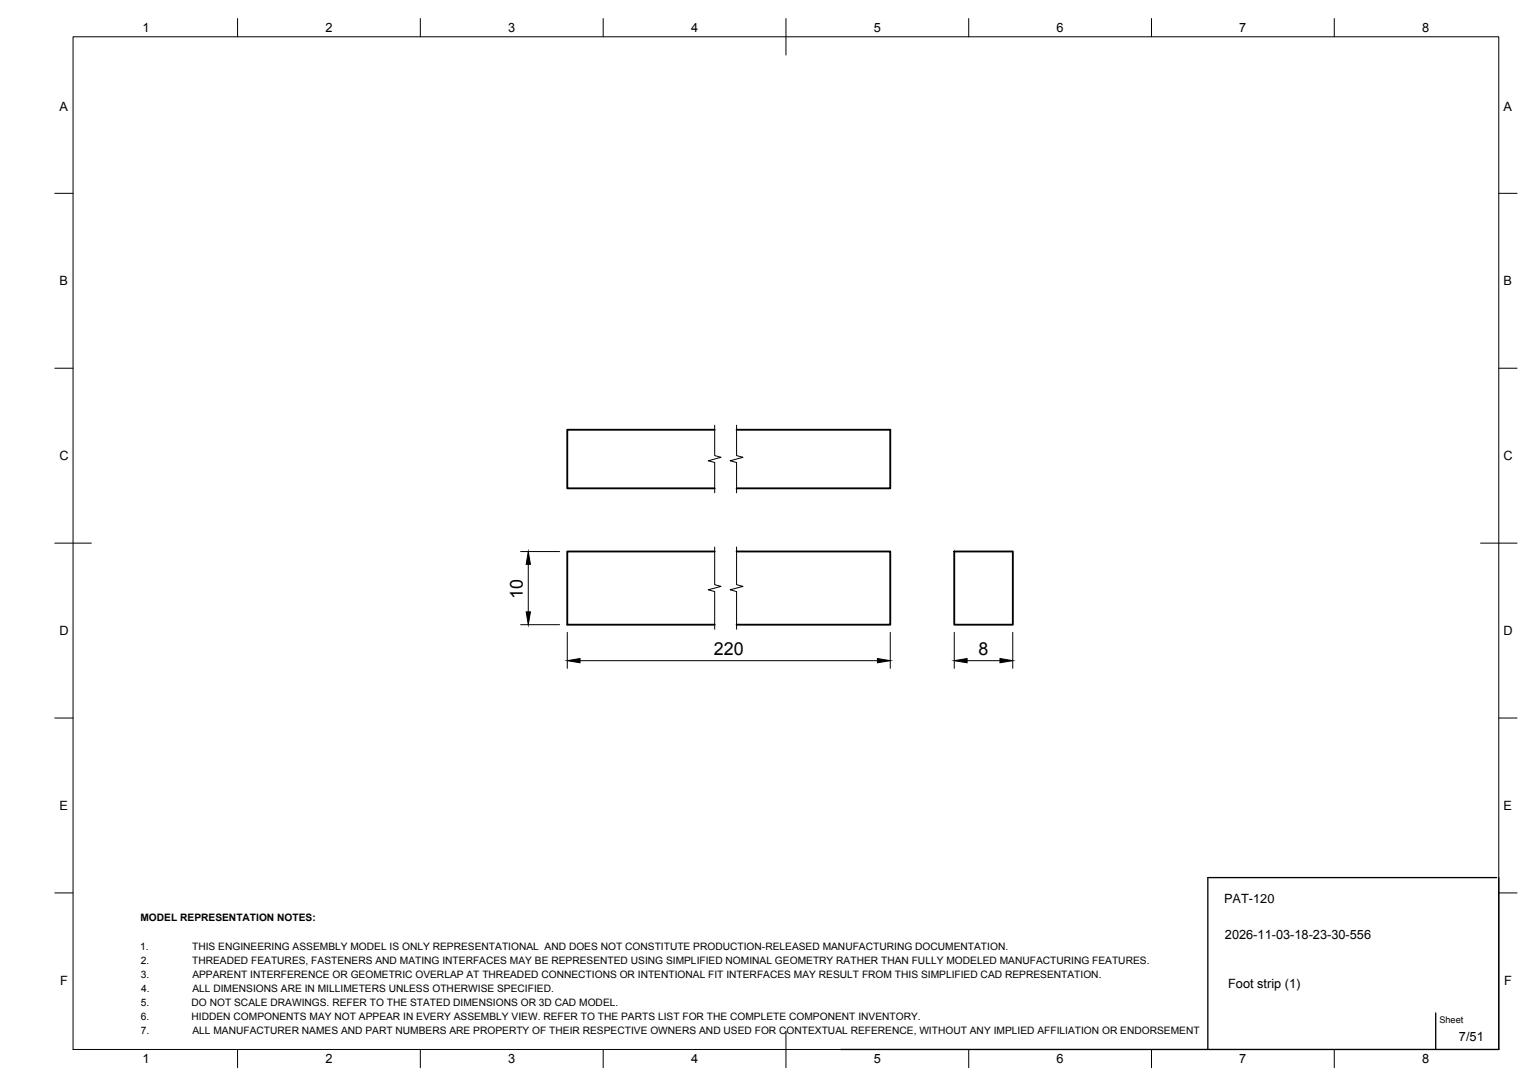
ISO-10303-21;
HEADER;
/* Generated by software containing ST-Developer
 * from STEP Tools, Inc. (www.steptools.com) 
 */

FILE_DESCRIPTION(
/* description */ ('Vibration shaker table dummy'),
/* implementation_level */ '2;1');

FILE_NAME(
/* name */ 'Foot strip (1).step',
/* time_stamp */ '2026-10-27T10:55:14-07:00',
/* author */ (''),
/* organization */ (''),
/* preprocessor_version */ 'ST-DEVELOPER v20.2',
/* originating_system */ 'Autodesk Translation Framework v15.17.0.0',
/* authorisation */ '');

FILE_SCHEMA (('AUTOMOTIVE_DESIGN { 1 0 10303 214 3 1 1 }'));
ENDSEC;

DATA;
#10=MECHANICAL_DESIGN_GEOMETRIC_PRESENTATION_REPRESENTATION('',(#688),#22394);
#596=SHAPE_REPRESENTATION_RELATIONSHIP('SRR','None',#22642,#642);
#642=ADVANCED_BREP_SHAPE_REPRESENTATION('',(#734),#22348);
#688=STYLED_ITEM('',(#22947),#734);
#734=MANIFOLD_SOLID_BREP('Body1',#9206);
#1072=PLANE('',#9843);
#1073=PLANE('',#9844);
#1074=PLANE('',#9845);
#1075=PLANE('',#9846);
#1076=PLANE('',#9847);
#1077=PLANE('',#9848);
#1375=FACE_OUTER_BOUND('',#1917,.T.);
#1376=FACE_OUTER_BOUND('',#1918,.T.);
#1377=FACE_OUTER_BOUND('',#1919,.T.);
#1378=FACE_OUTER_BOUND('',#1920,.T.);
#1379=FACE_OUTER_BOUND('',#1921,.T.);
#1380=FACE_OUTER_BOUND('',#1922,.T.);
#1917=EDGE_LOOP('',(#6426,#6427,#6428,#6429));
#1918=EDGE_LOOP('',(#6430,#6431,#6432,#6433));
#1919=EDGE_LOOP('',(#6434,#6435,#6436,#6437));
#1920=EDGE_LOOP('',(#6438,#6439,#6440,#6441));
#1921=EDGE_LOOP('',(#6442,#6443,#6444,#6445));
#1922=EDGE_LOOP('',(#6446,#6447,#6448,#6449));
#2668=LINE('',#14141,#3287);
#2669=LINE('',#14143,#3288);
#2670=LINE('',#14145,#3289);
#2671=LINE('',#14146,#3290);
#2672=LINE('',#14149,#3291);
#2673=LINE('',#14151,#3292);
#2674=LINE('',#14152,#3293);
#2675=LINE('',#14155,#3294);
#2676=LINE('',#14157,#3295);
#2677=LINE('',#14158,#3296);
#2678=LINE('',#14160,#3297);
#2679=LINE('',#14161,#3298);
#3287=VECTOR('',#11164,1.);
#3288=VECTOR('',#11165,1.);
#3289=VECTOR('',#11166,1.);
#3290=VECTOR('',#11167,1.);
#3291=VECTOR('',#11170,1.);
#3292=VECTOR('',#11171,1.);
#3293=VECTOR('',#11172,1.);
#3294=VECTOR('',#11175,1.);
#3295=VECTOR('',#11176,1.);
#3296=VECTOR('',#11177,1.);
#3297=VECTOR('',#11180,1.);
#3298=VECTOR('',#11181,1.);
#4427=VERTEX_POINT('',#14139);
#4428=VERTEX_POINT('',#14140);
#4429=VERTEX_POINT('',#14142);
#4430=VERTEX_POINT('',#14144);
#4431=VERTEX_POINT('',#14148);
#4432=VERTEX_POINT('',#14150);
#4433=VERTEX_POINT('',#14154);
#4434=VERTEX_POINT('',#14156);
#5206=EDGE_CURVE('',#4427,#4428,#2668,.T.);
#5207=EDGE_CURVE('',#4428,#4429,#2669,.T.);
#5208=EDGE_CURVE('',#4430,#4429,#2670,.T.);
#5209=EDGE_CURVE('',#4427,#4430,#2671,.T.);
#5210=EDGE_CURVE('',#4431,#4427,#2672,.T.);
#5211=EDGE_CURVE('',#4432,#4430,#2673,.T.);
#5212=EDGE_CURVE('',#4431,#4432,#2674,.T.);
#5213=EDGE_CURVE('',#4433,#4431,#2675,.T.);
#5214=EDGE_CURVE('',#4434,#4432,#2676,.T.);
#5215=EDGE_CURVE('',#4433,#4434,#2677,.T.);
#5216=EDGE_CURVE('',#4428,#4433,#2678,.T.);
#5217=EDGE_CURVE('',#4429,#4434,#2679,.T.);
#6426=ORIENTED_EDGE('',*,*,#5206,.T.);
#6427=ORIENTED_EDGE('',*,*,#5207,.T.);
#6428=ORIENTED_EDGE('',*,*,#5208,.F.);
#6429=ORIENTED_EDGE('',*,*,#5209,.F.);
#6430=ORIENTED_EDGE('',*,*,#5210,.T.);
#6431=ORIENTED_EDGE('',*,*,#5209,.T.);
#6432=ORIENTED_EDGE('',*,*,#5211,.F.);
#6433=ORIENTED_EDGE('',*,*,#5212,.F.);
#6434=ORIENTED_EDGE('',*,*,#5213,.T.);
#6435=ORIENTED_EDGE('',*,*,#5212,.T.);
#6436=ORIENTED_EDGE('',*,*,#5214,.F.);
#6437=ORIENTED_EDGE('',*,*,#5215,.F.);
#6438=ORIENTED_EDGE('',*,*,#5216,.T.);
#6439=ORIENTED_EDGE('',*,*,#5215,.T.);
#6440=ORIENTED_EDGE('',*,*,#5217,.F.);
#6441=ORIENTED_EDGE('',*,*,#5207,.F.);
#6442=ORIENTED_EDGE('',*,*,#5217,.T.);
#6443=ORIENTED_EDGE('',*,*,#5214,.T.);
#6444=ORIENTED_EDGE('',*,*,#5211,.T.);
#6445=ORIENTED_EDGE('',*,*,#5208,.T.);
#6446=ORIENTED_EDGE('',*,*,#5216,.F.);
#6447=ORIENTED_EDGE('',*,*,#5206,.F.);
#6448=ORIENTED_EDGE('',*,*,#5210,.F.);
#6449=ORIENTED_EDGE('',*,*,#5213,.F.);
#8740=ADVANCED_FACE('',(#1375),#1072,.T.);
#8741=ADVANCED_FACE('',(#1376),#1073,.T.);
#8742=ADVANCED_FACE('',(#1377),#1074,.T.);
#8743=ADVANCED_FACE('',(#1378),#1075,.T.);
#8744=ADVANCED_FACE('',(#1379),#1076,.T.);
#8745=ADVANCED_FACE('',(#1380),#1077,.F.);
#9206=CLOSED_SHELL('',(#8740,#8741,#8742,#8743,#8744,#8745));
#9842=AXIS2_PLACEMENT_3D('',#14137,#11160,#11161);
#9843=AXIS2_PLACEMENT_3D('',#14138,#11162,#11163);
#9844=AXIS2_PLACEMENT_3D('',#14147,#11168,#11169);
#9845=AXIS2_PLACEMENT_3D('',#14153,#11173,#11174);
#9846=AXIS2_PLACEMENT_3D('',#14159,#11178,#11179);
#9847=AXIS2_PLACEMENT_3D('',#14162,#11182,#11183);
#9848=AXIS2_PLACEMENT_3D('',#14163,#11184,#11185);
#11160=DIRECTION('axis',(0.,0.,1.));
#11161=DIRECTION('refdir',(1.,0.,0.));
#11162=DIRECTION('center_axis',(0.,1.,0.));
#11163=DIRECTION('ref_axis',(-1.,0.,0.));
#11164=DIRECTION('',(-1.,0.,0.));
#11165=DIRECTION('',(0.,0.,1.));
#11166=DIRECTION('',(-1.,0.,0.));
#11167=DIRECTION('',(0.,0.,1.));
#11168=DIRECTION('center_axis',(1.,0.,0.));
#11169=DIRECTION('ref_axis',(0.,1.,0.));
#11170=DIRECTION('',(0.,1.,0.));
#11171=DIRECTION('',(0.,1.,0.));
#11172=DIRECTION('',(0.,0.,1.));
#11173=DIRECTION('center_axis',(0.,-1.,0.));
#11174=DIRECTION('ref_axis',(1.,0.,0.));
#11175=DIRECTION('',(1.,0.,0.));
#11176=DIRECTION('',(1.,0.,0.));
#11177=DIRECTION('',(0.,0.,1.));
#11178=DIRECTION('center_axis',(-1.,0.,0.));
#11179=DIRECTION('ref_axis',(0.,-1.,0.));
#11180=DIRECTION('',(0.,-1.,0.));
#11181=DIRECTION('',(0.,-1.,0.));
#11182=DIRECTION('center_axis',(0.,0.,1.));
#11183=DIRECTION('ref_axis',(1.,0.,0.));
#11184=DIRECTION('center_axis',(0.,0.,1.));
#11185=DIRECTION('ref_axis',(1.,0.,0.));
#14137=CARTESIAN_POINT('',(0.,0.,0.));
#14138=CARTESIAN_POINT('Origin',(11.,12.5,-2.2));
#14139=CARTESIAN_POINT('',(11.,12.5,-2.2));
#14140=CARTESIAN_POINT('',(-11.,12.5,-2.2));
#14141=CARTESIAN_POINT('',(11.,12.5,-2.2));
#14142=CARTESIAN_POINT('',(-11.,12.5,-1.2));
#14143=CARTESIAN_POINT('',(-11.,12.5,-2.2));
#14144=CARTESIAN_POINT('',(11.,12.5,-1.2));
#14145=CARTESIAN_POINT('',(11.,12.5,-1.2));
#14146=CARTESIAN_POINT('',(11.,12.5,-2.2));
#14147=CARTESIAN_POINT('Origin',(11.,11.7,-2.2));
#14148=CARTESIAN_POINT('',(11.,11.7,-2.2));
#14149=CARTESIAN_POINT('',(11.,11.7,-2.2));
#14150=CARTESIAN_POINT('',(11.,11.7,-1.2));
#14151=CARTESIAN_POINT('',(11.,11.7,-1.2));
#14152=CARTESIAN_POINT('',(11.,11.7,-2.2));
#14153=CARTESIAN_POINT('Origin',(-11.,11.7,-2.2));
#14154=CARTESIAN_POINT('',(-11.,11.7,-2.2));
#14155=CARTESIAN_POINT('',(-11.,11.7,-2.2));
#14156=CARTESIAN_POINT('',(-11.,11.7,-1.2));
#14157=CARTESIAN_POINT('',(-11.,11.7,-1.2));
#14158=CARTESIAN_POINT('',(-11.,11.7,-2.2));
#14159=CARTESIAN_POINT('Origin',(-11.,12.5,-2.2));
#14160=CARTESIAN_POINT('',(-11.,12.5,-2.2));
#14161=CARTESIAN_POINT('',(-11.,12.5,-1.2));
#14162=CARTESIAN_POINT('Origin',(0.,12.1,-1.2));
#14163=CARTESIAN_POINT('Origin',(0.,12.1,-2.2));
#22297=UNCERTAINTY_MEASURE_WITH_UNIT(LENGTH_MEASURE(0.001),#22395,
'DISTANCE_ACCURACY_VALUE',
'Maximum model space distance between geometric entities at asserted c
onnectivities');
#22343=UNCERTAINTY_MEASURE_WITH_UNIT(LENGTH_MEASURE(0.001),#22395,
'DISTANCE_ACCURACY_VALUE',
'Maximum model space distance between geometric entities at asserted c
onnectivities');
#22348=(
GEOMETRIC_REPRESENTATION_CONTEXT(3)
GLOBAL_UNCERTAINTY_ASSIGNED_CONTEXT((#22297))
GLOBAL_UNIT_ASSIGNED_CONTEXT((#22395,#22397,#22398))
REPRESENTATION_CONTEXT('','3D')
);
#22394=(
GEOMETRIC_REPRESENTATION_CONTEXT(3)
GLOBAL_UNCERTAINTY_ASSIGNED_CONTEXT((#22343))
GLOBAL_UNIT_ASSIGNED_CONTEXT((#22395,#22397,#22398))
REPRESENTATION_CONTEXT('','3D')
);
#22395=(
LENGTH_UNIT()
NAMED_UNIT(*)
SI_UNIT(.CENTI.,.METRE.)
);
#22397=(
NAMED_UNIT(*)
PLANE_ANGLE_UNIT()
SI_UNIT($,.RADIAN.)
);
#22398=(
NAMED_UNIT(*)
SI_UNIT($,.STERADIAN.)
SOLID_ANGLE_UNIT()
);
#22403=SHAPE_DEFINITION_REPRESENTATION(#22453,#22642);
#22453=PRODUCT_DEFINITION_SHAPE('',$,#22693);
#22642=SHAPE_REPRESENTATION('',(#9842),#22348);
#22688=PRODUCT_DEFINITION_CONTEXT('part definition',#22840,'design');
#22693=PRODUCT_DEFINITION('Foot strip (1)','Foot strip (1)',#22743,#22688);
#22743=PRODUCT_DEFINITION_FORMATION('',$,#22846);
#22840=APPLICATION_CONTEXT(
'Core Data for Automotive Mechanical Design Process');
#22841=PRODUCT_CONTEXT('part definition',#22840,'mechanical');
#22846=PRODUCT('Foot strip (1)','Foot strip (1)','Foot strip (1)',(#22841));
#22941=COLOUR_RGB('Light Blue',0.38,0.62,0.78);
#22942=FILL_AREA_STYLE_COLOUR('',#22941);
#22943=FILL_AREA_STYLE('',(#22942));
#22944=SURFACE_STYLE_FILL_AREA(#22943);
#22945=SURFACE_SIDE_STYLE('',(#22944));
#22946=SURFACE_STYLE_USAGE(.BOTH.,#22945);
#22947=PRESENTATION_STYLE_ASSIGNMENT((#22946));
ENDSEC;
END-ISO-10303-21;
